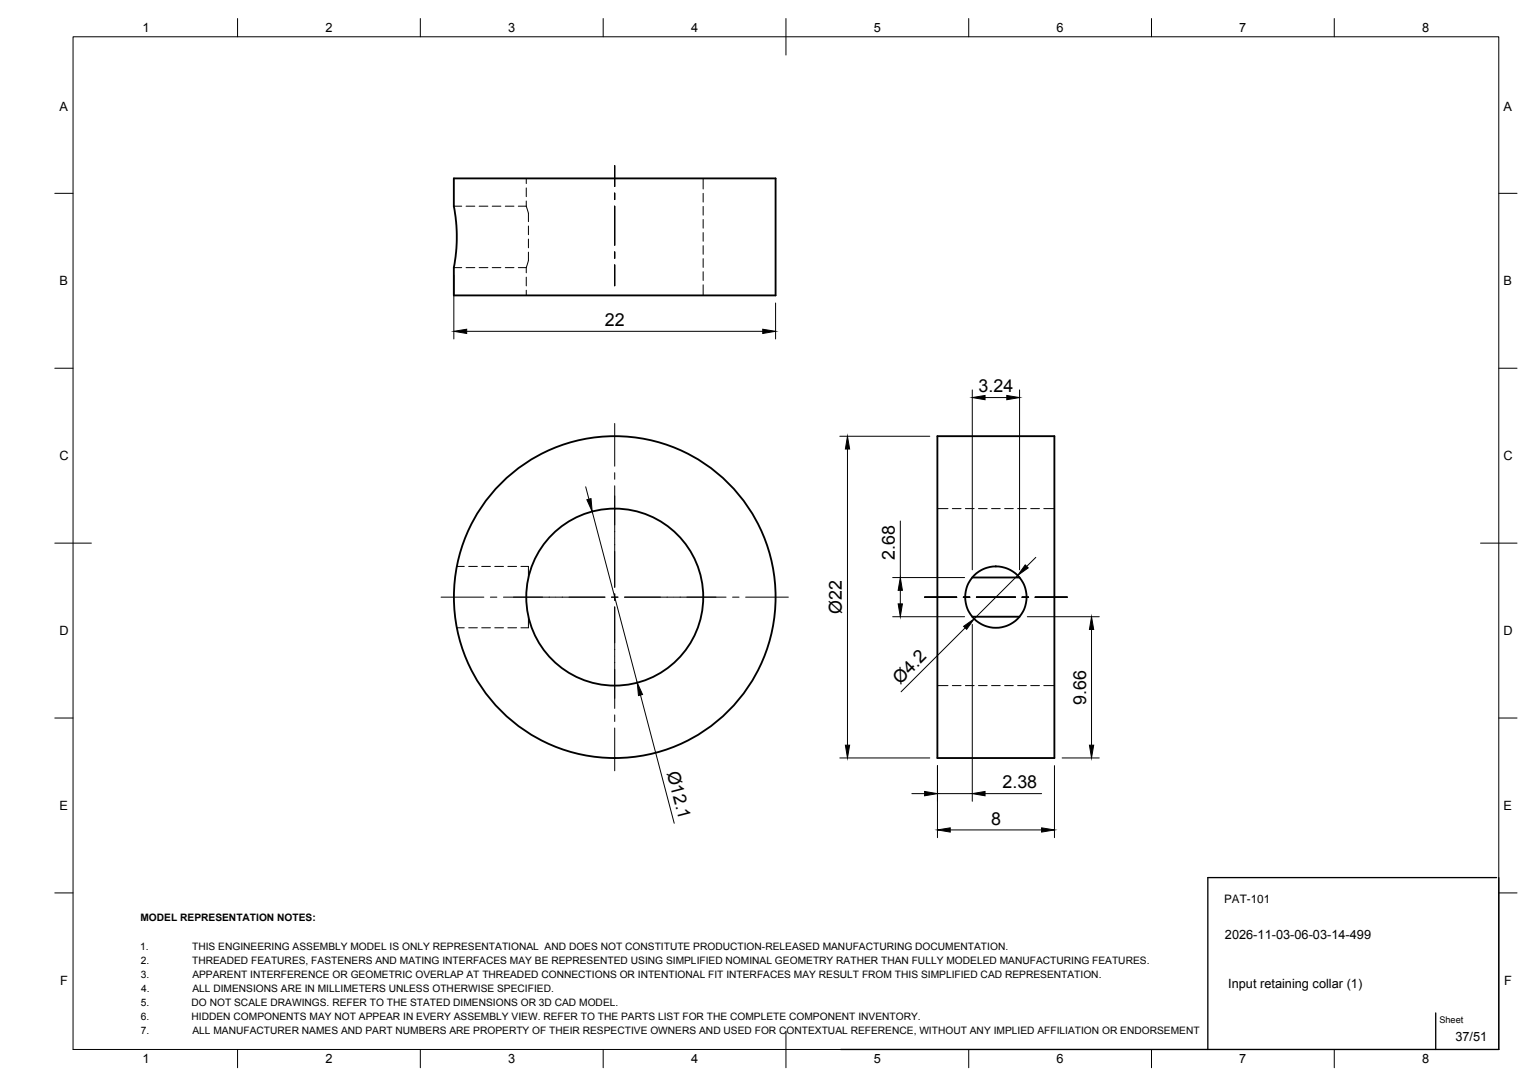
ISO-10303-21;
HEADER;
/* Generated by software containing ST-Developer
 * from STEP Tools, Inc. (www.steptools.com) 
 */

FILE_DESCRIPTION(
/* description */ ('Spur gear reduction stage 2-1 on bearing plates'),
/* implementation_level */ '2;1');

FILE_NAME(
/* name */ 'Input retaining collar (1).step',
/* time_stamp */ '2026-10-28T03:22:07-07:00',
/* author */ (''),
/* organization */ (''),
/* preprocessor_version */ 'ST-DEVELOPER v20.2',
/* originating_system */ 'Autodesk Translation Framework v15.17.0.0',
/* authorisation */ '');

FILE_SCHEMA (('AUTOMOTIVE_DESIGN { 1 0 10303 214 3 1 1 }'));
ENDSEC;

DATA;
#10=MECHANICAL_DESIGN_GEOMETRIC_PRESENTATION_REPRESENTATION('',(#991),#53909);
#703=B_SPLINE_CURVE_WITH_KNOTS('',3,(#18094,#18095,#18096,#18097,#18098,
#18099,#18100,#18101,#18102,#18103),.UNSPECIFIED.,.F.,.F.,(4,2,2,2,4),(0.818088904349169,
0.878131747417165,0.957937926194036,1.03774410497091,1.0977869480389),
 .UNSPECIFIED.);
#704=B_SPLINE_CURVE_WITH_KNOTS('',3,(#18109,#18110,#18111,#18112,#18113,
#18114,#18115,#18116,#18117,#18118,#18119,#18120,#18121,#18122,#18123,#18124,
#18125,#18126),.UNSPECIFIED.,.F.,.F.,(4,2,2,2,2,2,2,2,4),(0.,0.0793157643915219,
0.158631528783044,0.23794361593365,0.317255703084255,0.396567790234861,
0.475879877385467,0.555195641776989,0.634511406168511),.UNSPECIFIED.);
#705=B_SPLINE_CURVE_WITH_KNOTS('',3,(#18127,#18128,#18129,#18130,#18131,
#18132,#18133,#18134,#18135,#18136,#18137,#18138,#18139,#18140,#18141,#18142,
#18143,#18144),.UNSPECIFIED.,.F.,.F.,(4,2,2,2,2,2,2,2,4),(0.634511406168511,
0.713827170560033,0.793142934951554,0.87245502210216,0.951767109252766,
1.03107919640337,1.11039128355398,1.1897070479455,1.26902281233702),
 .UNSPECIFIED.);
#706=B_SPLINE_CURVE_WITH_KNOTS('',3,(#18147,#18148,#18149,#18150,#18151,
#18152,#18153,#18154,#18155,#18156),.UNSPECIFIED.,.F.,.F.,(4,2,2,2,4),(0.179463620219812,
0.239506463287808,0.319312642064679,0.399118820841549,0.459161663909545),
 .UNSPECIFIED.);
#890=SHAPE_REPRESENTATION_RELATIONSHIP('SRR','None',#54120,#933);
#933=ADVANCED_BREP_SHAPE_REPRESENTATION('',(#1046),#53894);
#991=STYLED_ITEM('',(#54383),#1046);
#1046=MANIFOLD_SOLID_BREP('Body1',#11318);
#1208=FACE_BOUND('',#2610,.T.);
#1209=FACE_BOUND('',#2612,.T.);
#1210=FACE_BOUND('',#2614,.T.);
#1211=FACE_BOUND('',#2616,.T.);
#1375=PLANE('',#12537);
#1376=PLANE('',#12542);
#1377=PLANE('',#12549);
#1378=PLANE('',#12550);
#1810=FACE_OUTER_BOUND('',#2606,.T.);
#1811=FACE_OUTER_BOUND('',#2607,.T.);
#1812=FACE_OUTER_BOUND('',#2608,.T.);
#1813=FACE_OUTER_BOUND('',#2609,.T.);
#1814=FACE_OUTER_BOUND('',#2611,.T.);
#1815=FACE_OUTER_BOUND('',#2613,.T.);
#1816=FACE_OUTER_BOUND('',#2615,.T.);
#2606=EDGE_LOOP('',(#8580,#8581));
#2607=EDGE_LOOP('',(#8582,#8583,#8584,#8585,#8586,#8587,#8588,#8589,#8590));
#2608=EDGE_LOOP('',(#8591,#8592,#8593));
#2609=EDGE_LOOP('',(#8594,#8595,#8596,#8597));
#2610=EDGE_LOOP('',(#8598,#8599,#8600,#8601));
#2611=EDGE_LOOP('',(#8602,#8603,#8604,#8605));
#2612=EDGE_LOOP('',(#8606,#8607));
#2613=EDGE_LOOP('',(#8608));
#2614=EDGE_LOOP('',(#8609));
#2615=EDGE_LOOP('',(#8610));
#2616=EDGE_LOOP('',(#8611));
#3215=LINE('',#18090,#3856);
#3216=LINE('',#18107,#3857);
#3217=LINE('',#18158,#3858);
#3218=LINE('',#18163,#3859);
#3219=LINE('',#18169,#3860);
#3856=VECTOR('',#14684,1.);
#3857=VECTOR('',#14691,0.21);
#3858=VECTOR('',#14696,1.);
#3859=VECTOR('',#14701,0.605);
#3860=VECTOR('',#14708,1.1);
#4599=CIRCLE('',#12538,0.21);
#4600=CIRCLE('',#12540,0.21);
#4601=CIRCLE('',#12541,0.21);
#4602=CIRCLE('',#12544,0.605);
#4603=CIRCLE('',#12545,0.605);
#4604=CIRCLE('',#12547,1.1);
#4605=CIRCLE('',#12548,1.1);
#5207=VERTEX_POINT('',#18088);
#5208=VERTEX_POINT('',#18089);
#5209=VERTEX_POINT('',#18093);
#5210=VERTEX_POINT('',#18104);
#5211=VERTEX_POINT('',#18106);
#5212=VERTEX_POINT('',#18108);
#5213=VERTEX_POINT('',#18145);
#5214=VERTEX_POINT('',#18160);
#5215=VERTEX_POINT('',#18162);
#5216=VERTEX_POINT('',#18166);
#5217=VERTEX_POINT('',#18168);
#6432=EDGE_CURVE('',#5207,#5208,#3215,.T.);
#6433=EDGE_CURVE('',#5207,#5208,#4599,.T.);
#6434=EDGE_CURVE('',#5209,#5207,#703,.T.);
#6435=EDGE_CURVE('',#5210,#5209,#4600,.T.);
#6436=EDGE_CURVE('',#5210,#5211,#3216,.T.);
#6437=EDGE_CURVE('',#5212,#5211,#704,.T.);
#6438=EDGE_CURVE('',#5211,#5212,#705,.T.);
#6439=EDGE_CURVE('',#5213,#5210,#4601,.T.);
#6440=EDGE_CURVE('',#5208,#5213,#706,.T.);
#6441=EDGE_CURVE('',#5213,#5209,#3217,.T.);
#6442=EDGE_CURVE('',#5214,#5214,#4602,.T.);
#6443=EDGE_CURVE('',#5214,#5215,#3218,.T.);
#6444=EDGE_CURVE('',#5215,#5215,#4603,.T.);
#6445=EDGE_CURVE('',#5216,#5216,#4604,.T.);
#6446=EDGE_CURVE('',#5216,#5217,#3219,.T.);
#6447=EDGE_CURVE('',#5217,#5217,#4605,.T.);
#8580=ORIENTED_EDGE('',*,*,#6432,.F.);
#8581=ORIENTED_EDGE('',*,*,#6433,.T.);
#8582=ORIENTED_EDGE('',*,*,#6434,.F.);
#8583=ORIENTED_EDGE('',*,*,#6435,.F.);
#8584=ORIENTED_EDGE('',*,*,#6436,.T.);
#8585=ORIENTED_EDGE('',*,*,#6437,.F.);
#8586=ORIENTED_EDGE('',*,*,#6438,.F.);
#8587=ORIENTED_EDGE('',*,*,#6436,.F.);
#8588=ORIENTED_EDGE('',*,*,#6439,.F.);
#8589=ORIENTED_EDGE('',*,*,#6440,.F.);
#8590=ORIENTED_EDGE('',*,*,#6433,.F.);
#8591=ORIENTED_EDGE('',*,*,#6441,.F.);
#8592=ORIENTED_EDGE('',*,*,#6439,.T.);
#8593=ORIENTED_EDGE('',*,*,#6435,.T.);
#8594=ORIENTED_EDGE('',*,*,#6442,.F.);
#8595=ORIENTED_EDGE('',*,*,#6443,.T.);
#8596=ORIENTED_EDGE('',*,*,#6444,.T.);
#8597=ORIENTED_EDGE('',*,*,#6443,.F.);
#8598=ORIENTED_EDGE('',*,*,#6440,.T.);
#8599=ORIENTED_EDGE('',*,*,#6441,.T.);
#8600=ORIENTED_EDGE('',*,*,#6434,.T.);
#8601=ORIENTED_EDGE('',*,*,#6432,.T.);
#8602=ORIENTED_EDGE('',*,*,#6445,.F.);
#8603=ORIENTED_EDGE('',*,*,#6446,.T.);
#8604=ORIENTED_EDGE('',*,*,#6447,.T.);
#8605=ORIENTED_EDGE('',*,*,#6446,.F.);
#8606=ORIENTED_EDGE('',*,*,#6437,.T.);
#8607=ORIENTED_EDGE('',*,*,#6438,.T.);
#8608=ORIENTED_EDGE('',*,*,#6445,.T.);
#8609=ORIENTED_EDGE('',*,*,#6442,.T.);
#8610=ORIENTED_EDGE('',*,*,#6447,.F.);
#8611=ORIENTED_EDGE('',*,*,#6444,.F.);
#10536=CYLINDRICAL_SURFACE('',#12539,0.21);
#10537=CYLINDRICAL_SURFACE('',#12543,0.605);
#10538=CYLINDRICAL_SURFACE('',#12546,1.1);
#10930=ADVANCED_FACE('',(#1810),#1375,.T.);
#10931=ADVANCED_FACE('',(#1811),#10536,.F.);
#10932=ADVANCED_FACE('',(#1812),#1376,.T.);
#10933=ADVANCED_FACE('',(#1813,#1208),#10537,.F.);
#10934=ADVANCED_FACE('',(#1814,#1209),#10538,.T.);
#10935=ADVANCED_FACE('',(#1815,#1210),#1377,.T.);
#10936=ADVANCED_FACE('',(#1816,#1211),#1378,.F.);
#11318=CLOSED_SHELL('',(#10930,#10931,#10932,#10933,#10934,#10935,#10936));
#12536=AXIS2_PLACEMENT_3D('',#18086,#14680,#14681);
#12537=AXIS2_PLACEMENT_3D('',#18087,#14682,#14683);
#12538=AXIS2_PLACEMENT_3D('',#18091,#14685,#14686);
#12539=AXIS2_PLACEMENT_3D('',#18092,#14687,#14688);
#12540=AXIS2_PLACEMENT_3D('',#18105,#14689,#14690);
#12541=AXIS2_PLACEMENT_3D('',#18146,#14692,#14693);
#12542=AXIS2_PLACEMENT_3D('',#18157,#14694,#14695);
#12543=AXIS2_PLACEMENT_3D('',#18159,#14697,#14698);
#12544=AXIS2_PLACEMENT_3D('',#18161,#14699,#14700);
#12545=AXIS2_PLACEMENT_3D('',#18164,#14702,#14703);
#12546=AXIS2_PLACEMENT_3D('',#18165,#14704,#14705);
#12547=AXIS2_PLACEMENT_3D('',#18167,#14706,#14707);
#12548=AXIS2_PLACEMENT_3D('',#18170,#14709,#14710);
#12549=AXIS2_PLACEMENT_3D('',#18171,#14711,#14712);
#12550=AXIS2_PLACEMENT_3D('',#18172,#14713,#14714);
#14680=DIRECTION('axis',(0.,0.,1.));
#14681=DIRECTION('refdir',(1.,0.,0.));
#14682=DIRECTION('center_axis',(0.,0.,1.));
#14683=DIRECTION('ref_axis',(1.,0.,0.));
#14684=DIRECTION('',(0.,1.,0.));
#14685=DIRECTION('center_axis',(0.,0.,1.));
#14686=DIRECTION('ref_axis',(1.,0.,0.));
#14687=DIRECTION('center_axis',(0.,0.,1.));
#14688=DIRECTION('ref_axis',(1.,0.,0.));
#14689=DIRECTION('center_axis',(0.,0.,1.));
#14690=DIRECTION('ref_axis',(1.,0.,0.));
#14691=DIRECTION('',(0.,0.,1.));
#14692=DIRECTION('center_axis',(0.,0.,1.));
#14693=DIRECTION('ref_axis',(1.,0.,0.));
#14694=DIRECTION('center_axis',(0.,0.,1.));
#14695=DIRECTION('ref_axis',(1.,0.,0.));
#14696=DIRECTION('',(0.,-1.,0.));
#14697=DIRECTION('center_axis',(0.,1.,0.));
#14698=DIRECTION('ref_axis',(1.,0.,0.));
#14699=DIRECTION('center_axis',(0.,-1.,0.));
#14700=DIRECTION('ref_axis',(1.,0.,0.));
#14701=DIRECTION('',(0.,-1.,0.));
#14702=DIRECTION('center_axis',(0.,-1.,0.));
#14703=DIRECTION('ref_axis',(1.,0.,0.));
#14704=DIRECTION('center_axis',(0.,1.,0.));
#14705=DIRECTION('ref_axis',(1.,0.,0.));
#14706=DIRECTION('center_axis',(0.,1.,0.));
#14707=DIRECTION('ref_axis',(1.,0.,0.));
#14708=DIRECTION('',(0.,-1.,0.));
#14709=DIRECTION('center_axis',(0.,1.,0.));
#14710=DIRECTION('ref_axis',(1.,0.,0.));
#14711=DIRECTION('center_axis',(0.,1.,0.));
#14712=DIRECTION('ref_axis',(1.,0.,0.));
#14713=DIRECTION('center_axis',(0.,1.,0.));
#14714=DIRECTION('ref_axis',(1.,0.,0.));
#18086=CARTESIAN_POINT('',(0.,0.,0.));
#18087=CARTESIAN_POINT('Origin',(0.,5.1,0.59));
#18088=CARTESIAN_POINT('',(0.133884278389959,4.93821310312637,0.59));
#18089=CARTESIAN_POINT('',(0.133884278389959,5.26178689687363,0.59));
#18090=CARTESIAN_POINT('',(0.133884278389959,4.7,0.59));
#18091=CARTESIAN_POINT('Origin',(0.,5.1,0.59));
#18092=CARTESIAN_POINT('Origin',(0.,5.1,0.59));
#18093=CARTESIAN_POINT('',(-0.133884278389959,4.93821310312637,0.59));
#18094=CARTESIAN_POINT('Ctrl Pts',(-0.133884278389959,4.93821310312636,
0.59));
#18095=CARTESIAN_POINT('Ctrl Pts',(-0.118254395260804,4.92527883178237,
0.59354677224418));
#18096=CARTESIAN_POINT('Ctrl Pts',(-0.1001097876823,4.91420068341256,0.596982247899573));
#18097=CARTESIAN_POINT('Ctrl Pts',(-0.0548298721325195,4.89536143894557,
0.603074162899704));
#18098=CARTESIAN_POINT('Ctrl Pts',(-0.0266020595922903,4.89,0.605));
#18099=CARTESIAN_POINT('Ctrl Pts',(0.0266020595922903,4.89,0.605));
#18100=CARTESIAN_POINT('Ctrl Pts',(0.0548298721325186,4.89536143894557,
0.603074162899704));
#18101=CARTESIAN_POINT('Ctrl Pts',(0.1001097876823,4.91420068341256,0.596982247899573));
#18102=CARTESIAN_POINT('Ctrl Pts',(0.118254395260804,4.92527883178237,0.59354677224418));
#18103=CARTESIAN_POINT('Ctrl Pts',(0.133884278389959,4.93821310312637,0.59));
#18104=CARTESIAN_POINT('',(-0.21,5.1,0.59));
#18105=CARTESIAN_POINT('Origin',(0.,5.1,0.59));
#18106=CARTESIAN_POINT('',(-0.21,5.1,1.07976849370594));
#18107=CARTESIAN_POINT('',(-0.21,5.1,0.59));
#18108=CARTESIAN_POINT('',(0.21,5.1,1.07976849370594));
#18109=CARTESIAN_POINT('Ctrl Pts',(0.21,5.1,1.07976849370594));
#18110=CARTESIAN_POINT('Ctrl Pts',(0.21,5.07356141186949,1.07976849370594));
#18111=CARTESIAN_POINT('Ctrl Pts',(0.204702922670977,5.04540621874507,1.08084015664674));
#18112=CARTESIAN_POINT('Ctrl Pts',(0.183251796806355,4.99368655445866,1.08468313707126));
#18113=CARTESIAN_POINT('Ctrl Pts',(0.167101177357215,4.97011632925886,1.08739593054622));
#18114=CARTESIAN_POINT('Ctrl Pts',(0.129884533480965,4.93289968538261,1.09246633289124));
#18115=CARTESIAN_POINT('Ctrl Pts',(0.106313940757289,4.91674838983659,1.09515738895358));
#18116=CARTESIAN_POINT('Ctrl Pts',(0.0545930033295209,4.89529677343026,
1.09895039220591));
#18117=CARTESIAN_POINT('Ctrl Pts',(0.0264373623835353,4.89,1.1));
#18118=CARTESIAN_POINT('Ctrl Pts',(-0.0264373623835352,4.89,1.1));
#18119=CARTESIAN_POINT('Ctrl Pts',(-0.0545930033295208,4.89529677343026,
1.09895039220591));
#18120=CARTESIAN_POINT('Ctrl Pts',(-0.106313940757289,4.91674838983659,
1.09515738895358));
#18121=CARTESIAN_POINT('Ctrl Pts',(-0.129884533480965,4.93289968538261,
1.09246633289124));
#18122=CARTESIAN_POINT('Ctrl Pts',(-0.167101177357215,4.97011632925886,
1.08739593054622));
#18123=CARTESIAN_POINT('Ctrl Pts',(-0.183251796806354,4.99368655445866,
1.08468313707126));
#18124=CARTESIAN_POINT('Ctrl Pts',(-0.204702922670976,5.04540621874507,
1.08084015664674));
#18125=CARTESIAN_POINT('Ctrl Pts',(-0.21,5.07356141186949,1.07976849370594));
#18126=CARTESIAN_POINT('Ctrl Pts',(-0.21,5.1,1.07976849370594));
#18127=CARTESIAN_POINT('Ctrl Pts',(-0.21,5.1,1.07976849370594));
#18128=CARTESIAN_POINT('Ctrl Pts',(-0.21,5.12643858813051,1.07976849370594));
#18129=CARTESIAN_POINT('Ctrl Pts',(-0.204702922670977,5.15459378125493,
1.08084015664674));
#18130=CARTESIAN_POINT('Ctrl Pts',(-0.183251796806355,5.20631344554134,
1.08468313707126));
#18131=CARTESIAN_POINT('Ctrl Pts',(-0.167101177357215,5.22988367074114,
1.08739593054622));
#18132=CARTESIAN_POINT('Ctrl Pts',(-0.129884533480965,5.26710031461738,
1.09246633289124));
#18133=CARTESIAN_POINT('Ctrl Pts',(-0.106313940757289,5.28325161016341,
1.09515738895358));
#18134=CARTESIAN_POINT('Ctrl Pts',(-0.0545930033295209,5.30470322656974,
1.09895039220591));
#18135=CARTESIAN_POINT('Ctrl Pts',(-0.0264373623835353,5.31,1.1));
#18136=CARTESIAN_POINT('Ctrl Pts',(0.0264373623835353,5.31,1.1));
#18137=CARTESIAN_POINT('Ctrl Pts',(0.0545930033295212,5.30470322656974,
1.09895039220591));
#18138=CARTESIAN_POINT('Ctrl Pts',(0.106313940757289,5.28325161016341,1.09515738895358));
#18139=CARTESIAN_POINT('Ctrl Pts',(0.129884533480965,5.26710031461738,1.09246633289124));
#18140=CARTESIAN_POINT('Ctrl Pts',(0.167101177357214,5.22988367074114,1.08739593054622));
#18141=CARTESIAN_POINT('Ctrl Pts',(0.183251796806355,5.20631344554134,1.08468313707126));
#18142=CARTESIAN_POINT('Ctrl Pts',(0.204702922670977,5.15459378125493,1.08084015664674));
#18143=CARTESIAN_POINT('Ctrl Pts',(0.21,5.12643858813051,1.07976849370594));
#18144=CARTESIAN_POINT('Ctrl Pts',(0.21,5.1,1.07976849370594));
#18145=CARTESIAN_POINT('',(-0.133884278389959,5.26178689687363,0.59));
#18146=CARTESIAN_POINT('Origin',(0.,5.1,0.59));
#18147=CARTESIAN_POINT('Ctrl Pts',(0.133884278389959,5.26178689687363,0.59));
#18148=CARTESIAN_POINT('Ctrl Pts',(0.118254395260804,5.27472116821763,0.59354677224418));
#18149=CARTESIAN_POINT('Ctrl Pts',(0.1001097876823,5.28579931658744,0.596982247899573));
#18150=CARTESIAN_POINT('Ctrl Pts',(0.0548298721325194,5.30463856105443,
0.603074162899704));
#18151=CARTESIAN_POINT('Ctrl Pts',(0.0266020595922903,5.31,0.605));
#18152=CARTESIAN_POINT('Ctrl Pts',(-0.0266020595922903,5.31,0.605));
#18153=CARTESIAN_POINT('Ctrl Pts',(-0.0548298721325194,5.30463856105443,
0.603074162899704));
#18154=CARTESIAN_POINT('Ctrl Pts',(-0.1001097876823,5.28579931658744,0.596982247899573));
#18155=CARTESIAN_POINT('Ctrl Pts',(-0.118254395260804,5.27472116821763,
0.59354677224418));
#18156=CARTESIAN_POINT('Ctrl Pts',(-0.133884278389958,5.26178689687363,
0.59));
#18157=CARTESIAN_POINT('Origin',(0.,5.1,0.59));
#18158=CARTESIAN_POINT('',(-0.133884278389959,4.7,0.59));
#18159=CARTESIAN_POINT('Origin',(0.,4.7,0.));
#18160=CARTESIAN_POINT('',(-0.605,5.5,7.40911313484149E-17));
#18161=CARTESIAN_POINT('Origin',(0.,5.5,0.));
#18162=CARTESIAN_POINT('',(-0.605,4.7,7.40911313484149E-17));
#18163=CARTESIAN_POINT('',(-0.605,4.7,7.40911313484149E-17));
#18164=CARTESIAN_POINT('Origin',(0.,4.7,0.));
#18165=CARTESIAN_POINT('Origin',(0.,4.7,0.));
#18166=CARTESIAN_POINT('',(-1.1,5.5,1.34711147906209E-16));
#18167=CARTESIAN_POINT('Origin',(0.,5.5,0.));
#18168=CARTESIAN_POINT('',(-1.1,4.7,1.34711147906209E-16));
#18169=CARTESIAN_POINT('',(-1.1,4.7,1.34711147906209E-16));
#18170=CARTESIAN_POINT('Origin',(0.,4.7,0.));
#18171=CARTESIAN_POINT('Origin',(0.,5.5,0.));
#18172=CARTESIAN_POINT('Origin',(0.,4.7,0.));
#53844=UNCERTAINTY_MEASURE_WITH_UNIT(LENGTH_MEASURE(0.001),#53910,
'DISTANCE_ACCURACY_VALUE',
'Maximum model space distance between geometric entities at asserted c
onnectivities');
#53859=UNCERTAINTY_MEASURE_WITH_UNIT(LENGTH_MEASURE(0.001),#53910,
'DISTANCE_ACCURACY_VALUE',
'Maximum model space distance between geometric entities at asserted c
onnectivities');
#53894=(
GEOMETRIC_REPRESENTATION_CONTEXT(3)
GLOBAL_UNCERTAINTY_ASSIGNED_CONTEXT((#53844))
GLOBAL_UNIT_ASSIGNED_CONTEXT((#53910,#53912,#53913))
REPRESENTATION_CONTEXT('','3D')
);
#53909=(
GEOMETRIC_REPRESENTATION_CONTEXT(3)
GLOBAL_UNCERTAINTY_ASSIGNED_CONTEXT((#53859))
GLOBAL_UNIT_ASSIGNED_CONTEXT((#53910,#53912,#53913))
REPRESENTATION_CONTEXT('','3D')
);
#53910=(
LENGTH_UNIT()
NAMED_UNIT(*)
SI_UNIT(.CENTI.,.METRE.)
);
#53912=(
NAMED_UNIT(*)
PLANE_ANGLE_UNIT()
SI_UNIT($,.RADIAN.)
);
#53913=(
NAMED_UNIT(*)
SI_UNIT($,.STERADIAN.)
SOLID_ANGLE_UNIT()
);
#53948=SHAPE_DEFINITION_REPRESENTATION(#54046,#54120);
#54046=PRODUCT_DEFINITION_SHAPE('',$,#54170);
#54120=SHAPE_REPRESENTATION('',(#12536),#53894);
#54135=PRODUCT_DEFINITION_CONTEXT('part definition',#54284,'design');
#54170=PRODUCT_DEFINITION('Input retaining collar (1)',
'Input retaining collar (1)',#54219,#54135);
#54219=PRODUCT_DEFINITION_FORMATION('',$,#54320);
#54284=APPLICATION_CONTEXT(
'Core Data for Automotive Mechanical Design Process');
#54285=PRODUCT_CONTEXT('part definition',#54284,'mechanical');
#54320=PRODUCT('Input retaining collar (1)','Input retaining collar (1)',
'Input retaining collar (1)',(#54285));
#54377=COLOUR_RGB('Light Blue',0.38,0.62,0.78);
#54378=FILL_AREA_STYLE_COLOUR('',#54377);
#54379=FILL_AREA_STYLE('',(#54378));
#54380=SURFACE_STYLE_FILL_AREA(#54379);
#54381=SURFACE_SIDE_STYLE('',(#54380));
#54382=SURFACE_STYLE_USAGE(.BOTH.,#54381);
#54383=PRESENTATION_STYLE_ASSIGNMENT((#54382));
ENDSEC;
END-ISO-10303-21;
